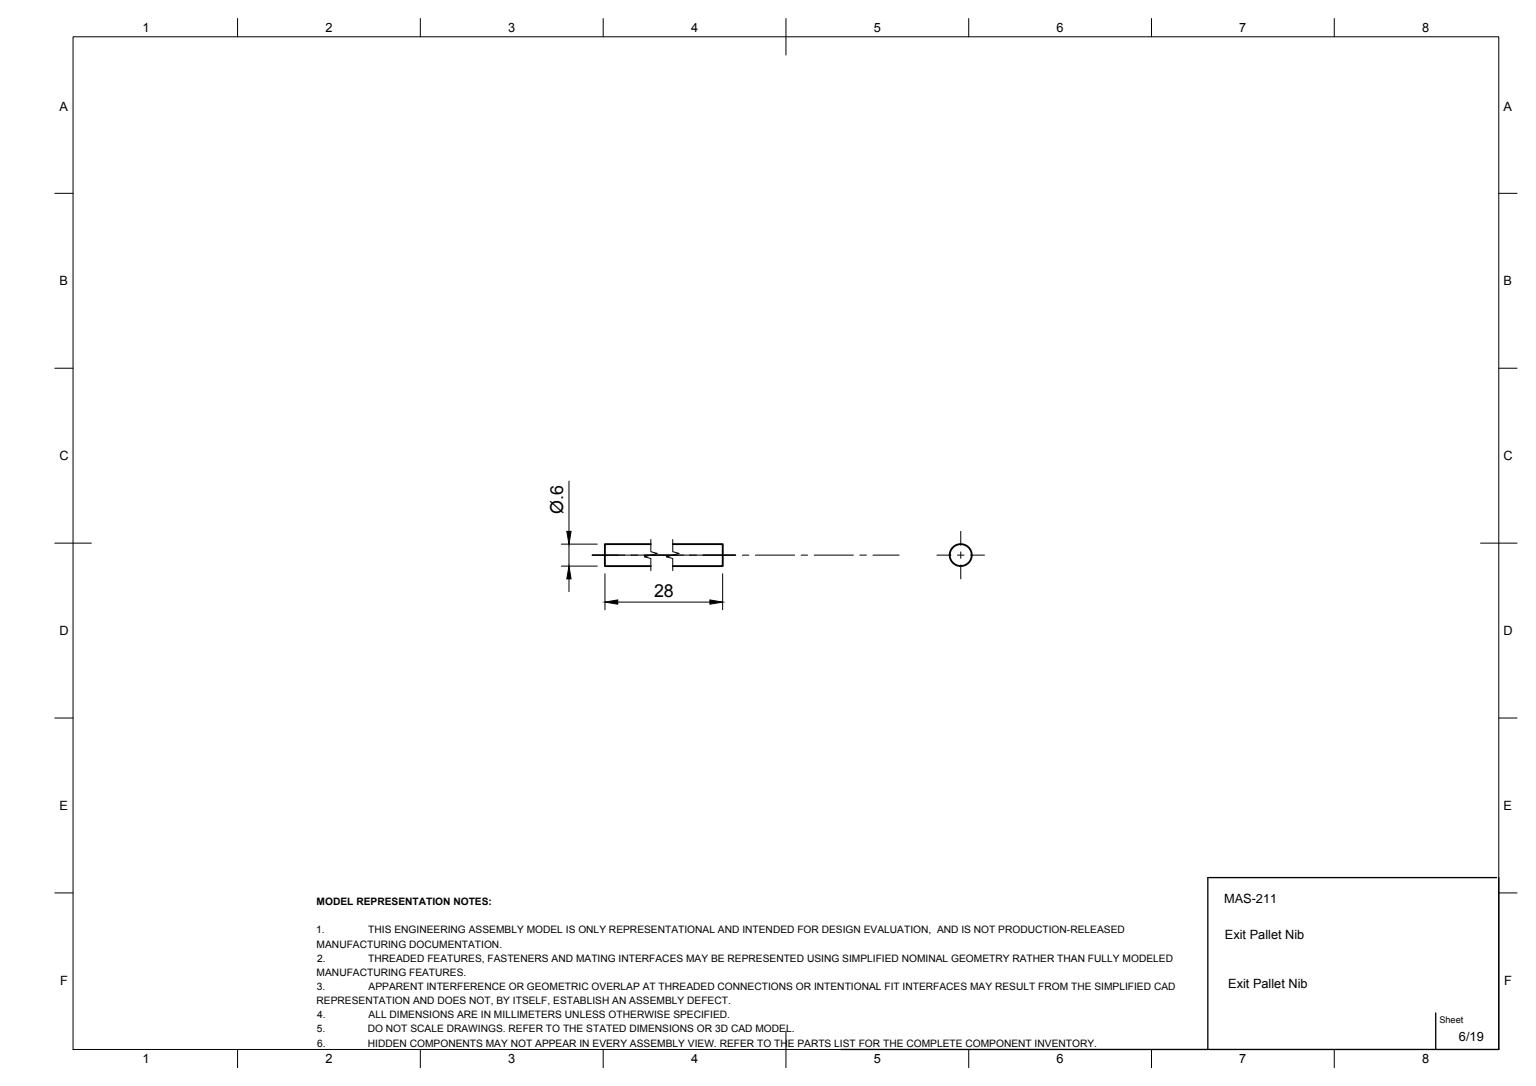
ISO-10303-21;
HEADER;
FILE_DESCRIPTION(
 (''),
 '2;1');
FILE_NAME ( 'Exit Pallet Nib.step', '2026-10-05T20:07:59+06:00', ( '' ), ( '' ), 'STEP AP214', 'Unspecified', '' );
FILE_SCHEMA (('AUTOMOTIVE_DESIGN { 1 0 10303 214 3 1 1 }'));
ENDSEC;
DATA;
#10=MECHANICAL_DESIGN_GEOMETRIC_PRESENTATION_REPRESENTATION('',(#322),#196741);
#322=STYLED_ITEM('',(#196765),#341) ;
#341=MANIFOLD_SOLID_BREP('Exit Pallet Nib',#8718) ;
#367=PLANE('',#8803) ;
#368=PLANE('',#8804) ;
#629=CIRCLE('',#8801,0.300000000000005) ;
#630=CIRCLE('',#8802,0.3) ;
#915=FACE_OUTER_BOUND('',#1398,.T.) ;
#916=FACE_OUTER_BOUND('',#1399,.T.) ;
#917=FACE_OUTER_BOUND('',#1400,.T.) ;
#1398=EDGE_LOOP('',(#5896,#5897,#5898,#5899)) ;
#1399=EDGE_LOOP('',(#5900)) ;
#1400=EDGE_LOOP('',(#5901)) ;
#1905=LINE('',#79309,#2608) ;
#2608=VECTOR('',#9609,0.300000000000007) ;
#3559=VERTEX_POINT('',#79306) ;
#3560=VERTEX_POINT('',#79308) ;
#4456=EDGE_CURVE('',#3559,#3559,#629,.T.) ;
#4457=EDGE_CURVE('',#3559,#3560,#1905,.T.) ;
#4458=EDGE_CURVE('',#3560,#3560,#630,.T.) ;
#5896=ORIENTED_EDGE('',*,*,#4456,.T.) ;
#5897=ORIENTED_EDGE('',*,*,#4457,.T.) ;
#5898=ORIENTED_EDGE('',*,*,#4458,.F.) ;
#5899=ORIENTED_EDGE('',*,*,#4457,.F.) ;
#5900=ORIENTED_EDGE('',*,*,#4458,.T.) ;
#5901=ORIENTED_EDGE('',*,*,#4456,.F.) ;
#8143=CYLINDRICAL_SURFACE('',#8800,0.300000000000007) ;
#8298=ADVANCED_FACE('',(#915),#8143,.T.) ;
#8299=ADVANCED_FACE('',(#916),#367,.T.) ;
#8300=ADVANCED_FACE('',(#917),#368,.T.) ;
#8718=CLOSED_SHELL('',(#8298,#8299,#8300)) ;
#8800=AXIS2_PLACEMENT_3D('',#79305,#9605,#9606) ;
#8801=AXIS2_PLACEMENT_3D('',#79307,#9607,#9608) ;
#8802=AXIS2_PLACEMENT_3D('',#79310,#9610,#9611) ;
#8803=AXIS2_PLACEMENT_3D('',#79311,#9612,#9613) ;
#8804=AXIS2_PLACEMENT_3D('',#79312,#9614,#9615) ;
#9605=DIRECTION('center_axis',(0.946101641249535,-1.74835062554578E-30,
0.323869857234255)) ;
#9606=DIRECTION('ref_axis',(0.,1.,0.)) ;
#9607=DIRECTION('center_axis',(-0.946101641249527,2.48640733553338E-14,
-0.323869857234278)) ;
#9608=DIRECTION('ref_axis',(0.188203553203274,-0.813826036051078,-0.549787782337014)) ;
#9609=DIRECTION('',(-0.946101641249535,1.74835062554578E-30,-0.323869857234255)) ;
#9610=DIRECTION('center_axis',(-0.946101641249534,-2.31955132725112E-15,
-0.323869857234258)) ;
#9611=DIRECTION('ref_axis',(0.188203553203289,-0.813826036051069,-0.549787782337023)) ;
#9612=DIRECTION('center_axis',(-0.946101641249535,1.97215226305253E-31,
-0.323869857234254)) ;
#9613=DIRECTION('ref_axis',(-0.323869857234254,0.,0.946101641249535)) ;
#9614=DIRECTION('center_axis',(0.946101641249535,0.,0.323869857234254)) ;
#9615=DIRECTION('ref_axis',(0.323869857234254,0.,-0.946101641249535)) ;
#79305=CARTESIAN_POINT('Origin',(22.7064337521429,-12.,137.828896526385)) ;
#79306=CARTESIAN_POINT('',(3.78440092715221,-12.3,131.3514993817)) ;
#79307=CARTESIAN_POINT('Origin',(3.7844009271522,-12.,131.3514993817)) ;
#79308=CARTESIAN_POINT('',(-22.7064450278348,-12.3,122.283143379141)) ;
#79309=CARTESIAN_POINT('',(22.7064337521429,-12.3,137.828896526385)) ;
#79310=CARTESIAN_POINT('Origin',(-22.7064450278348,-12.,122.283143379141)) ;
#79311=CARTESIAN_POINT('Origin',(-22.7064450278348,-12.3,122.283143379141)) ;
#79312=CARTESIAN_POINT('Origin',(3.78440656499815,14.,131.351482912198)) ;
#196737=UNCERTAINTY_MEASURE_WITH_UNIT(LENGTH_MEASURE(0.01),#196742,
'DISTANCE_ACCURACY_VALUE',
'Maximum model space distance between geometric entities at asserted c
onnectivities') ;
#196738=UNCERTAINTY_MEASURE_WITH_UNIT(LENGTH_MEASURE(0.01),#196742,
'DISTANCE_ACCURACY_VALUE',
'Maximum model space distance between geometric entities at asserted c
onnectivities') ;
#196740=(
GEOMETRIC_REPRESENTATION_CONTEXT(3)
GLOBAL_UNCERTAINTY_ASSIGNED_CONTEXT((#196737))
GLOBAL_UNIT_ASSIGNED_CONTEXT((#196742,#196744,#196745))
REPRESENTATION_CONTEXT('','3D')
) ;
#196741=(
GEOMETRIC_REPRESENTATION_CONTEXT(3)
GLOBAL_UNCERTAINTY_ASSIGNED_CONTEXT((#196738))
GLOBAL_UNIT_ASSIGNED_CONTEXT((#196742,#196744,#196745))
REPRESENTATION_CONTEXT('','3D')
) ;
#196742=(
LENGTH_UNIT()
NAMED_UNIT(*)
SI_UNIT(.MILLI.,.METRE.)
) ;
#196744=(
NAMED_UNIT(*)
PLANE_ANGLE_UNIT()
SI_UNIT($,.RADIAN.)
) ;
#196745=(
NAMED_UNIT(*)
SI_UNIT($,.STERADIAN.)
SOLID_ANGLE_UNIT()
) ;
#196753=PRODUCT_DEFINITION_CONTEXT('part definition',#196761,'design') ;
#196761=APPLICATION_CONTEXT(
'Core Data for Automotive Mechanical Design Process') ;
#196762=PRODUCT_CONTEXT('part definition',#196761,'mechanical') ;
#196765=PRESENTATION_STYLE_ASSIGNMENT((#196767)) ;
#196767=SURFACE_STYLE_USAGE(.BOTH.,#196769) ;
#196769=SURFACE_SIDE_STYLE('',(#196771)) ;
#196771=SURFACE_STYLE_FILL_AREA(#196773) ;
#196773=FILL_AREA_STYLE('Steel - Satin',(#196775)) ;
#196775=FILL_AREA_STYLE_COLOUR('Steel - Satin',#196777) ;
#196777=COLOUR_RGB('Steel - Satin', 0.09019608, 0.27058824, 0.51372549) ;
#196851=CARTESIAN_POINT ( '', ( 0.0, 0.0, 0.0 ) ) ;
#196852=DIRECTION ( '', ( 0.0, 0.0, 1.0 ) ) ;
#196853=DIRECTION ( '', ( 1.0, 0.0, 0.0 ) ) ;
#196854=AXIS2_PLACEMENT_3D ( '', #196851, #196852, #196853 ) ;
#196855=ADVANCED_BREP_SHAPE_REPRESENTATION ( 'Exit Pallet Nib', ( #341, #196854, #196865, #197277 ), #196740 ) ;
#196856=PRODUCT( 'Exit Pallet Nib', 'Exit Pallet Nib', '', ( #196762 ) ) ;
#196857=PRODUCT_DEFINITION_FORMATION ( '', '', #196856 ) ;
#196858=PRODUCT_DEFINITION( 'Exit Pallet Nib', 'Exit Pallet Nib', #196857, #196753 ) ;
#196859=PRODUCT_DEFINITION_SHAPE ( '', '', #196858 ) ;
#196860=SHAPE_DEFINITION_REPRESENTATION ( #196859, #196855 ) ;
#196862=CARTESIAN_POINT ( '', ( 0.0, 0.0, 0.0 ) ) ;
#196863=DIRECTION ( '', ( 0.0, 0.0, 1.0 ) ) ;
#196864=DIRECTION ( '', ( 1.0, 0.0, 0.0 ) ) ;
#196865=AXIS2_PLACEMENT_3D ( '', #196862, #196863, #196864 ) ;
#197274=CARTESIAN_POINT ( '', ( 0.0, 0.0, 0.0 ) ) ;
#197275=DIRECTION ( '', ( 0.0, 0.0, 1.0 ) ) ;
#197276=DIRECTION ( '', ( 1.0, 0.0, 0.0 ) ) ;
#197277=AXIS2_PLACEMENT_3D ( '', #197274, #197275, #197276 ) ;
ENDSEC;
END-ISO-10303-21;
